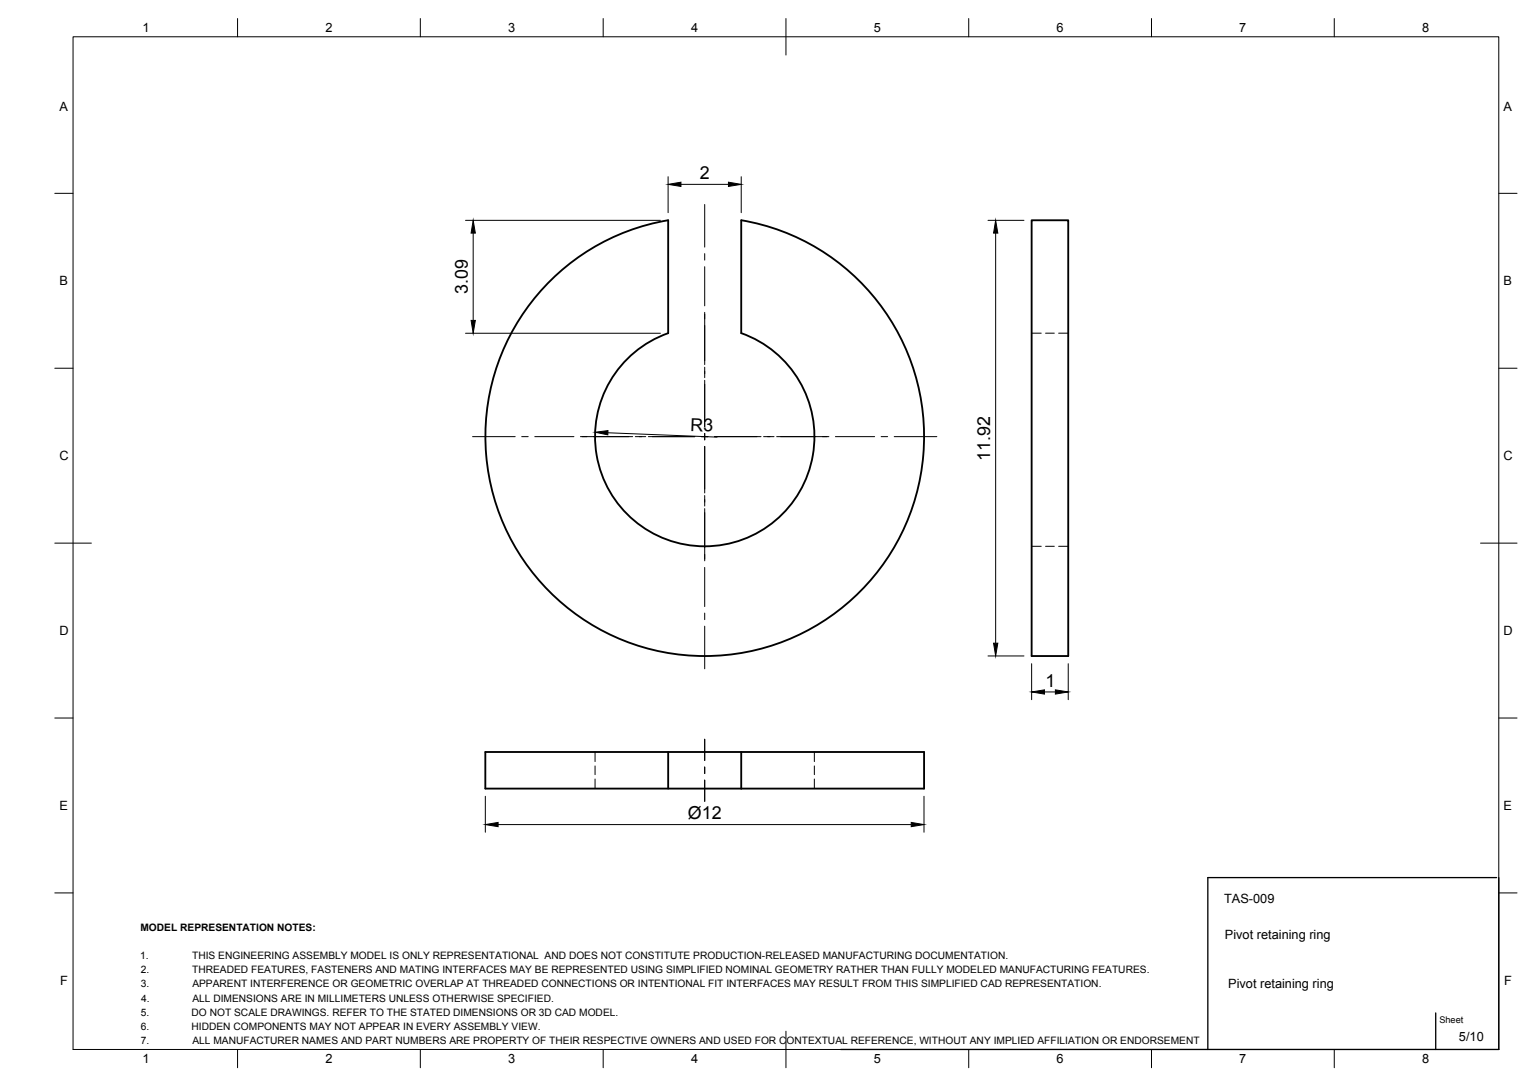
ISO-10303-21;
HEADER;
/* Generated by software containing ST-Developer
 * from STEP Tools, Inc. (www.steptools.com) 
 */

FILE_DESCRIPTION(
/* description */ (''),
/* implementation_level */ '2;1');

FILE_NAME(
/* name */ 'Pivot retaining ring.step',
/* time_stamp */ '2026-11-12T00:53:40-08:00',
/* author */ (''),
/* organization */ (''),
/* preprocessor_version */ 'ST-DEVELOPER v20.2',
/* originating_system */ 'Autodesk Translation Framework v15.17.0.0',
/* authorisation */ '');

FILE_SCHEMA (('AUTOMOTIVE_DESIGN { 1 0 10303 214 3 1 1 }'));
ENDSEC;

DATA;
#10=MECHANICAL_DESIGN_GEOMETRIC_PRESENTATION_REPRESENTATION('',(#574),#22129);
#556=SHAPE_REPRESENTATION_RELATIONSHIP('SRR','None',#22175,#565);
#565=ADVANCED_BREP_SHAPE_REPRESENTATION('',(#583),#22121);
#574=STYLED_ITEM('',(#22234),#583);
#583=MANIFOLD_SOLID_BREP('Body1',#8805);
#785=PLANE('',#9077);
#786=PLANE('',#9078);
#787=PLANE('',#9079);
#788=PLANE('',#9086);
#1046=FACE_OUTER_BOUND('',#1538,.T.);
#1047=FACE_OUTER_BOUND('',#1539,.T.);
#1048=FACE_OUTER_BOUND('',#1540,.T.);
#1049=FACE_OUTER_BOUND('',#1541,.T.);
#1050=FACE_OUTER_BOUND('',#1542,.T.);
#1051=FACE_OUTER_BOUND('',#1543,.T.);
#1538=EDGE_LOOP('',(#6462,#6463,#6464,#6465));
#1539=EDGE_LOOP('',(#6466,#6467,#6468,#6469));
#1540=EDGE_LOOP('',(#6470,#6471,#6472,#6473));
#1541=EDGE_LOOP('',(#6474,#6475,#6476,#6477));
#1542=EDGE_LOOP('',(#6478,#6479,#6480,#6481));
#1543=EDGE_LOOP('',(#6482,#6483,#6484,#6485));
#2320=LINE('',#12236,#3050);
#2321=LINE('',#12238,#3051);
#2322=LINE('',#12240,#3052);
#2323=LINE('',#12241,#3053);
#2324=LINE('',#12245,#3054);
#2325=LINE('',#12247,#3055);
#2326=LINE('',#12249,#3056);
#2327=LINE('',#12250,#3057);
#3050=VECTOR('',#10222,1.);
#3051=VECTOR('',#10223,1.);
#3052=VECTOR('',#10224,1.);
#3053=VECTOR('',#10225,1.);
#3054=VECTOR('',#10228,1.);
#3055=VECTOR('',#10229,1.);
#3056=VECTOR('',#10230,1.);
#3057=VECTOR('',#10231,1.);
#3408=CIRCLE('',#9080,0.6);
#3409=CIRCLE('',#9081,0.3);
#3410=CIRCLE('',#9083,0.3);
#3411=CIRCLE('',#9085,0.6);
#3820=VERTEX_POINT('',#12234);
#3821=VERTEX_POINT('',#12235);
#3822=VERTEX_POINT('',#12237);
#3823=VERTEX_POINT('',#12239);
#3824=VERTEX_POINT('',#12243);
#3825=VERTEX_POINT('',#12244);
#3826=VERTEX_POINT('',#12246);
#3827=VERTEX_POINT('',#12248);
#4784=EDGE_CURVE('',#3820,#3821,#2320,.T.);
#4785=EDGE_CURVE('',#3822,#3820,#2321,.T.);
#4786=EDGE_CURVE('',#3823,#3822,#2322,.T.);
#4787=EDGE_CURVE('',#3821,#3823,#2323,.T.);
#4788=EDGE_CURVE('',#3824,#3825,#2324,.T.);
#4789=EDGE_CURVE('',#3826,#3824,#2325,.T.);
#4790=EDGE_CURVE('',#3827,#3826,#2326,.T.);
#4791=EDGE_CURVE('',#3825,#3827,#2327,.T.);
#4792=EDGE_CURVE('',#3822,#3827,#3408,.T.);
#4793=EDGE_CURVE('',#3825,#3820,#3409,.T.);
#4794=EDGE_CURVE('',#3824,#3821,#3410,.T.);
#4795=EDGE_CURVE('',#3823,#3826,#3411,.T.);
#6462=ORIENTED_EDGE('',*,*,#4784,.F.);
#6463=ORIENTED_EDGE('',*,*,#4785,.F.);
#6464=ORIENTED_EDGE('',*,*,#4786,.F.);
#6465=ORIENTED_EDGE('',*,*,#4787,.F.);
#6466=ORIENTED_EDGE('',*,*,#4788,.F.);
#6467=ORIENTED_EDGE('',*,*,#4789,.F.);
#6468=ORIENTED_EDGE('',*,*,#4790,.F.);
#6469=ORIENTED_EDGE('',*,*,#4791,.F.);
#6470=ORIENTED_EDGE('',*,*,#4791,.T.);
#6471=ORIENTED_EDGE('',*,*,#4792,.F.);
#6472=ORIENTED_EDGE('',*,*,#4785,.T.);
#6473=ORIENTED_EDGE('',*,*,#4793,.F.);
#6474=ORIENTED_EDGE('',*,*,#4788,.T.);
#6475=ORIENTED_EDGE('',*,*,#4793,.T.);
#6476=ORIENTED_EDGE('',*,*,#4784,.T.);
#6477=ORIENTED_EDGE('',*,*,#4794,.F.);
#6478=ORIENTED_EDGE('',*,*,#4790,.T.);
#6479=ORIENTED_EDGE('',*,*,#4795,.F.);
#6480=ORIENTED_EDGE('',*,*,#4786,.T.);
#6481=ORIENTED_EDGE('',*,*,#4792,.T.);
#6482=ORIENTED_EDGE('',*,*,#4789,.T.);
#6483=ORIENTED_EDGE('',*,*,#4794,.T.);
#6484=ORIENTED_EDGE('',*,*,#4787,.T.);
#6485=ORIENTED_EDGE('',*,*,#4795,.T.);
#8195=CYLINDRICAL_SURFACE('',#9082,0.3);
#8196=CYLINDRICAL_SURFACE('',#9084,0.6);
#8463=ADVANCED_FACE('',(#1046),#785,.F.);
#8464=ADVANCED_FACE('',(#1047),#786,.F.);
#8465=ADVANCED_FACE('',(#1048),#787,.F.);
#8466=ADVANCED_FACE('',(#1049),#8195,.F.);
#8467=ADVANCED_FACE('',(#1050),#8196,.T.);
#8468=ADVANCED_FACE('',(#1051),#788,.T.);
#8805=CLOSED_SHELL('',(#8463,#8464,#8465,#8466,#8467,#8468));
#9076=AXIS2_PLACEMENT_3D('',#12232,#10218,#10219);
#9077=AXIS2_PLACEMENT_3D('',#12233,#10220,#10221);
#9078=AXIS2_PLACEMENT_3D('',#12242,#10226,#10227);
#9079=AXIS2_PLACEMENT_3D('',#12251,#10232,#10233);
#9080=AXIS2_PLACEMENT_3D('',#12252,#10234,#10235);
#9081=AXIS2_PLACEMENT_3D('',#12253,#10236,#10237);
#9082=AXIS2_PLACEMENT_3D('',#12254,#10238,#10239);
#9083=AXIS2_PLACEMENT_3D('',#12255,#10240,#10241);
#9084=AXIS2_PLACEMENT_3D('',#12256,#10242,#10243);
#9085=AXIS2_PLACEMENT_3D('',#12257,#10244,#10245);
#9086=AXIS2_PLACEMENT_3D('',#12258,#10246,#10247);
#10218=DIRECTION('axis',(0.,0.,1.));
#10219=DIRECTION('refdir',(1.,0.,0.));
#10220=DIRECTION('center_axis',(-1.,0.,0.));
#10221=DIRECTION('ref_axis',(0.,1.,0.));
#10222=DIRECTION('',(0.,0.,1.));
#10223=DIRECTION('',(0.,-1.,0.));
#10224=DIRECTION('',(0.,0.,-1.));
#10225=DIRECTION('',(0.,1.,0.));
#10226=DIRECTION('center_axis',(1.,0.,0.));
#10227=DIRECTION('ref_axis',(0.,-1.,0.));
#10228=DIRECTION('',(0.,0.,-1.));
#10229=DIRECTION('',(0.,-1.,0.));
#10230=DIRECTION('',(0.,0.,1.));
#10231=DIRECTION('',(0.,1.,0.));
#10232=DIRECTION('center_axis',(0.,0.,1.));
#10233=DIRECTION('ref_axis',(1.,0.,0.));
#10234=DIRECTION('center_axis',(0.,0.,1.));
#10235=DIRECTION('ref_axis',(1.,0.,0.));
#10236=DIRECTION('center_axis',(0.,0.,-1.));
#10237=DIRECTION('ref_axis',(1.,0.,0.));
#10238=DIRECTION('center_axis',(0.,0.,1.));
#10239=DIRECTION('ref_axis',(6.12323399573677E-17,-1.,0.));
#10240=DIRECTION('center_axis',(0.,0.,-1.));
#10241=DIRECTION('ref_axis',(1.,0.,0.));
#10242=DIRECTION('center_axis',(0.,0.,1.));
#10243=DIRECTION('ref_axis',(6.12323399573677E-17,-1.,0.));
#10244=DIRECTION('center_axis',(0.,0.,1.));
#10245=DIRECTION('ref_axis',(1.,0.,0.));
#10246=DIRECTION('center_axis',(0.,0.,1.));
#10247=DIRECTION('ref_axis',(1.,0.,0.));
#12232=CARTESIAN_POINT('',(0.,0.,0.));
#12233=CARTESIAN_POINT('Origin',(-0.1,0.,0.1));
#12234=CARTESIAN_POINT('',(-0.1,0.282842712474619,0.));
#12235=CARTESIAN_POINT('',(-0.1,0.282842712474619,0.1));
#12236=CARTESIAN_POINT('',(-0.1,0.282842712474619,0.));
#12237=CARTESIAN_POINT('',(-0.1,0.591607978309962,0.));
#12238=CARTESIAN_POINT('',(-0.1,0.,0.));
#12239=CARTESIAN_POINT('',(-0.1,0.591607978309962,0.1));
#12240=CARTESIAN_POINT('',(-0.1,0.591607978309962,0.));
#12241=CARTESIAN_POINT('',(-0.1,0.,0.1));
#12242=CARTESIAN_POINT('Origin',(0.1,1.2,0.1));
#12243=CARTESIAN_POINT('',(0.1,0.282842712474619,0.1));
#12244=CARTESIAN_POINT('',(0.1,0.282842712474619,0.));
#12245=CARTESIAN_POINT('',(0.1,0.282842712474619,0.));
#12246=CARTESIAN_POINT('',(0.1,0.591607978309962,0.1));
#12247=CARTESIAN_POINT('',(0.1,0.6,0.1));
#12248=CARTESIAN_POINT('',(0.1,0.591607978309962,0.));
#12249=CARTESIAN_POINT('',(0.1,0.591607978309962,0.));
#12250=CARTESIAN_POINT('',(0.1,0.6,0.));
#12251=CARTESIAN_POINT('Origin',(0.,0.,0.));
#12252=CARTESIAN_POINT('Origin',(0.,0.,0.));
#12253=CARTESIAN_POINT('Origin',(0.,0.,0.));
#12254=CARTESIAN_POINT('Origin',(0.,0.,0.));
#12255=CARTESIAN_POINT('Origin',(0.,0.,0.1));
#12256=CARTESIAN_POINT('Origin',(0.,0.,0.));
#12257=CARTESIAN_POINT('Origin',(0.,0.,0.1));
#12258=CARTESIAN_POINT('Origin',(0.,0.,0.1));
#22109=UNCERTAINTY_MEASURE_WITH_UNIT(LENGTH_MEASURE(0.001),#22130,
'DISTANCE_ACCURACY_VALUE',
'Maximum model space distance between geometric entities at asserted c
onnectivities');
#22117=UNCERTAINTY_MEASURE_WITH_UNIT(LENGTH_MEASURE(0.001),#22130,
'DISTANCE_ACCURACY_VALUE',
'Maximum model space distance between geometric entities at asserted c
onnectivities');
#22121=(
GEOMETRIC_REPRESENTATION_CONTEXT(3)
GLOBAL_UNCERTAINTY_ASSIGNED_CONTEXT((#22109))
GLOBAL_UNIT_ASSIGNED_CONTEXT((#22130,#22132,#22133))
REPRESENTATION_CONTEXT('','3D')
);
#22129=(
GEOMETRIC_REPRESENTATION_CONTEXT(3)
GLOBAL_UNCERTAINTY_ASSIGNED_CONTEXT((#22117))
GLOBAL_UNIT_ASSIGNED_CONTEXT((#22130,#22132,#22133))
REPRESENTATION_CONTEXT('','3D')
);
#22130=(
LENGTH_UNIT()
NAMED_UNIT(*)
SI_UNIT(.CENTI.,.METRE.)
);
#22132=(
NAMED_UNIT(*)
PLANE_ANGLE_UNIT()
SI_UNIT($,.RADIAN.)
);
#22133=(
NAMED_UNIT(*)
SI_UNIT($,.STERADIAN.)
SOLID_ANGLE_UNIT()
);
#22137=SHAPE_DEFINITION_REPRESENTATION(#22148,#22175);
#22148=PRODUCT_DEFINITION_SHAPE('',$,#22187);
#22175=SHAPE_REPRESENTATION('',(#9076),#22121);
#22183=PRODUCT_DEFINITION_CONTEXT('part definition',#22218,'design');
#22187=PRODUCT_DEFINITION('Pivot retaining ring','Pivot retaining ring',
#22198,#22183);
#22198=PRODUCT_DEFINITION_FORMATION('',$,#22223);
#22218=APPLICATION_CONTEXT(
'Core Data for Automotive Mechanical Design Process');
#22219=PRODUCT_CONTEXT('part definition',#22218,'mechanical');
#22223=PRODUCT('Pivot retaining ring','Pivot retaining ring',$,(#22219));
#22234=PRESENTATION_STYLE_ASSIGNMENT((#22242));
#22242=SURFACE_STYLE_USAGE(.BOTH.,#22250);
#22250=SURFACE_SIDE_STYLE('',(#22258));
#22258=SURFACE_STYLE_FILL_AREA(#22266);
#22266=FILL_AREA_STYLE('Dark gray',(#22274));
#22274=FILL_AREA_STYLE_COLOUR('Dark gray',#22282);
#22282=COLOUR_RGB('Dark gray',0.250980392156863,0.282352941176471,0.32156862745098);
ENDSEC;
END-ISO-10303-21;
